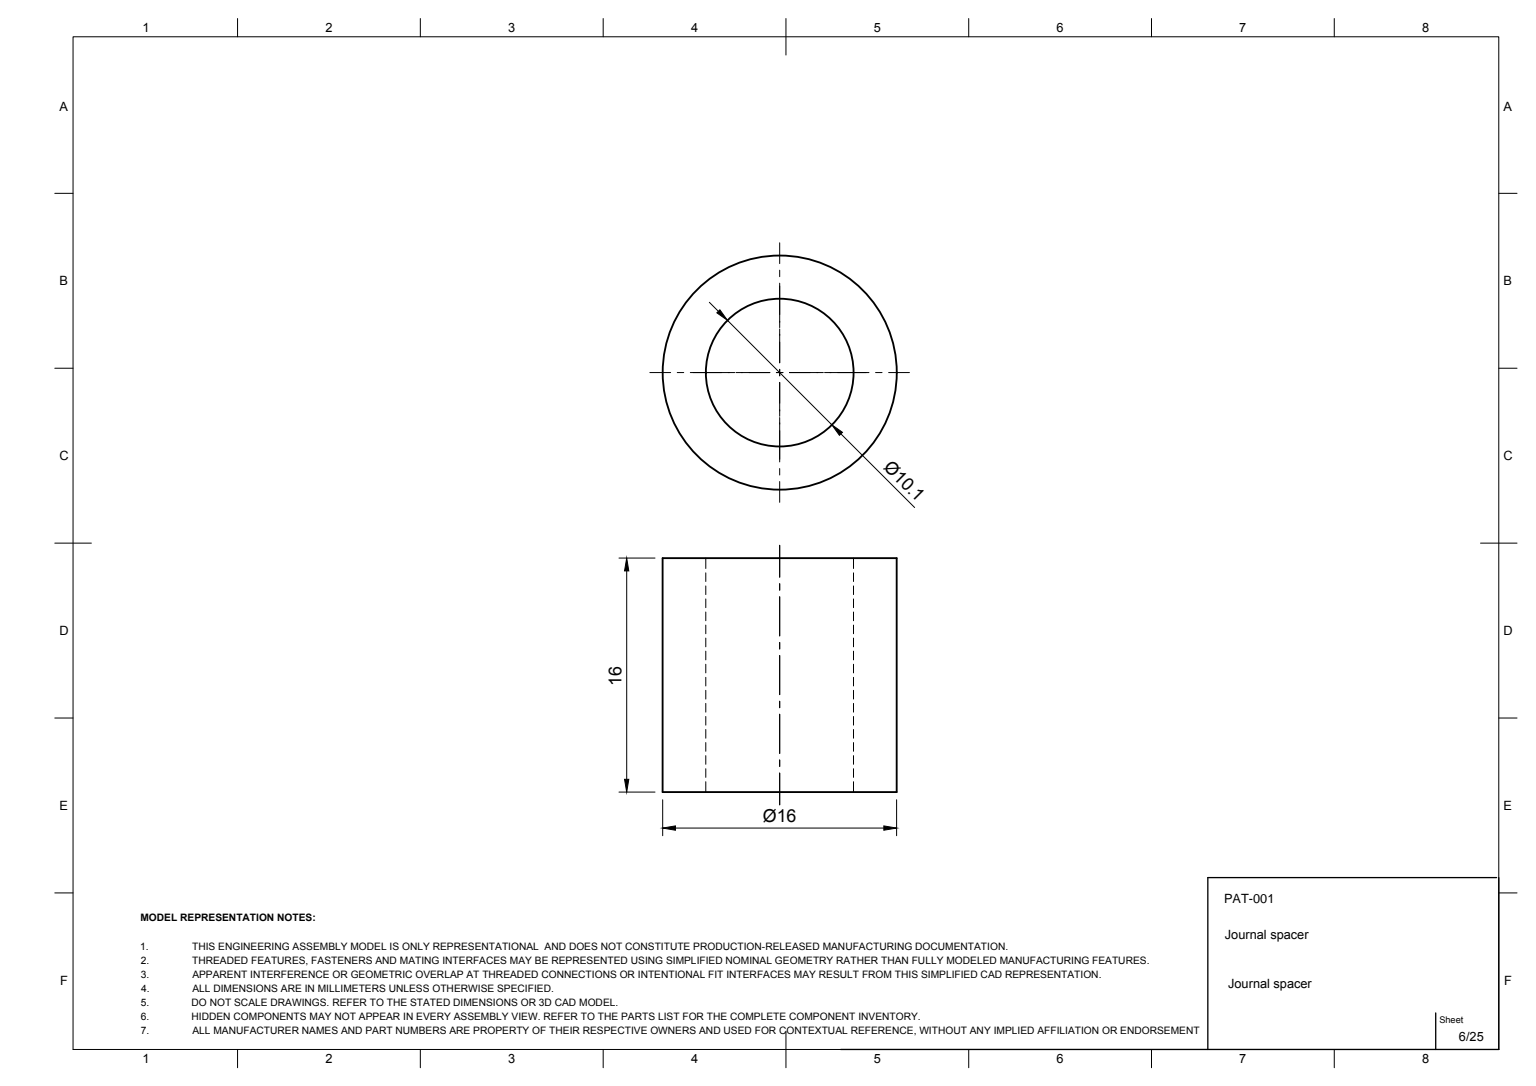
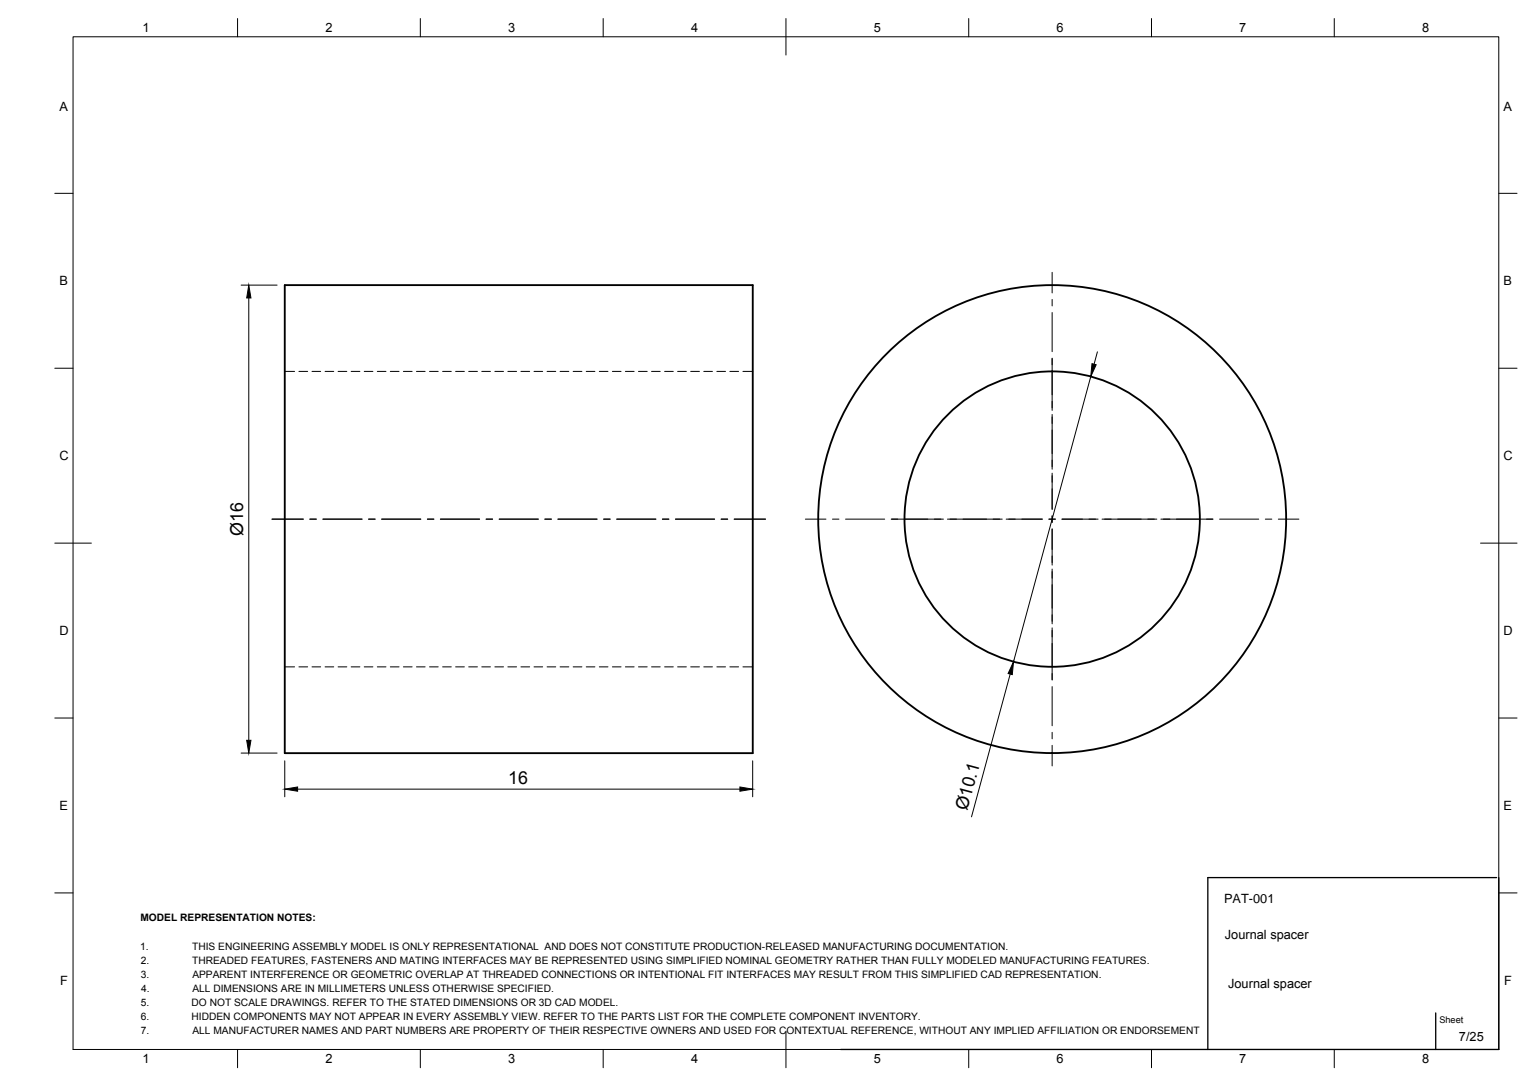
ISO-10303-21;
HEADER;
/* Generated by software containing ST-Developer
 * from STEP Tools, Inc. (www.steptools.com) 
 */

FILE_DESCRIPTION(
/* description */ ('PAT-001'),
/* implementation_level */ '2;1');

FILE_NAME(
/* name */ 'Journal spacer.step',
/* time_stamp */ '2026-10-29T17:07:15-07:00',
/* author */ (''),
/* organization */ (''),
/* preprocessor_version */ 'ST-DEVELOPER v20.2',
/* originating_system */ 'Autodesk Translation Framework v15.17.0.0',
/* authorisation */ '');

FILE_SCHEMA (('AUTOMOTIVE_DESIGN { 1 0 10303 214 3 1 1 }'));
ENDSEC;

DATA;
#10=MECHANICAL_DESIGN_GEOMETRIC_PRESENTATION_REPRESENTATION('',(#374),#9622);
#324=SHAPE_REPRESENTATION_RELATIONSHIP('SRR','None',#9747,#349);
#349=ADVANCED_BREP_SHAPE_REPRESENTATION('',(#407),#9596);
#374=STYLED_ITEM('',(#9955),#407);
#407=MANIFOLD_SOLID_BREP('Body1',#5199);
#441=FACE_BOUND('',#1029,.T.);
#442=FACE_BOUND('',#1031,.T.);
#534=PLANE('',#5540);
#535=PLANE('',#5541);
#726=FACE_OUTER_BOUND('',#1026,.T.);
#727=FACE_OUTER_BOUND('',#1027,.T.);
#728=FACE_OUTER_BOUND('',#1028,.T.);
#729=FACE_OUTER_BOUND('',#1030,.T.);
#1026=EDGE_LOOP('',(#3547,#3548,#3549,#3550));
#1027=EDGE_LOOP('',(#3551,#3552,#3553,#3554));
#1028=EDGE_LOOP('',(#3555));
#1029=EDGE_LOOP('',(#3556));
#1030=EDGE_LOOP('',(#3557));
#1031=EDGE_LOOP('',(#3558));
#1403=LINE('',#7752,#1808);
#1404=LINE('',#7758,#1809);
#1808=VECTOR('',#6166,0.505);
#1809=VECTOR('',#6173,0.8);
#2218=CIRCLE('',#5535,0.505);
#2219=CIRCLE('',#5536,0.505);
#2220=CIRCLE('',#5538,0.8);
#2221=CIRCLE('',#5539,0.8);
#2430=VERTEX_POINT('',#7749);
#2431=VERTEX_POINT('',#7751);
#2432=VERTEX_POINT('',#7755);
#2433=VERTEX_POINT('',#7757);
#2877=EDGE_CURVE('',#2430,#2430,#2218,.T.);
#2878=EDGE_CURVE('',#2430,#2431,#1403,.T.);
#2879=EDGE_CURVE('',#2431,#2431,#2219,.T.);
#2880=EDGE_CURVE('',#2432,#2432,#2220,.T.);
#2881=EDGE_CURVE('',#2432,#2433,#1404,.T.);
#2882=EDGE_CURVE('',#2433,#2433,#2221,.T.);
#3547=ORIENTED_EDGE('',*,*,#2877,.F.);
#3548=ORIENTED_EDGE('',*,*,#2878,.T.);
#3549=ORIENTED_EDGE('',*,*,#2879,.T.);
#3550=ORIENTED_EDGE('',*,*,#2878,.F.);
#3551=ORIENTED_EDGE('',*,*,#2880,.F.);
#3552=ORIENTED_EDGE('',*,*,#2881,.T.);
#3553=ORIENTED_EDGE('',*,*,#2882,.T.);
#3554=ORIENTED_EDGE('',*,*,#2881,.F.);
#3555=ORIENTED_EDGE('',*,*,#2880,.T.);
#3556=ORIENTED_EDGE('',*,*,#2877,.T.);
#3557=ORIENTED_EDGE('',*,*,#2882,.F.);
#3558=ORIENTED_EDGE('',*,*,#2879,.F.);
#4832=CYLINDRICAL_SURFACE('',#5534,0.505);
#4833=CYLINDRICAL_SURFACE('',#5537,0.8);
#4913=ADVANCED_FACE('',(#726),#4832,.F.);
#4914=ADVANCED_FACE('',(#727),#4833,.T.);
#4915=ADVANCED_FACE('',(#728,#441),#534,.T.);
#4916=ADVANCED_FACE('',(#729,#442),#535,.F.);
#5199=CLOSED_SHELL('',(#4913,#4914,#4915,#4916));
#5533=AXIS2_PLACEMENT_3D('',#7747,#6160,#6161);
#5534=AXIS2_PLACEMENT_3D('',#7748,#6162,#6163);
#5535=AXIS2_PLACEMENT_3D('',#7750,#6164,#6165);
#5536=AXIS2_PLACEMENT_3D('',#7753,#6167,#6168);
#5537=AXIS2_PLACEMENT_3D('',#7754,#6169,#6170);
#5538=AXIS2_PLACEMENT_3D('',#7756,#6171,#6172);
#5539=AXIS2_PLACEMENT_3D('',#7759,#6174,#6175);
#5540=AXIS2_PLACEMENT_3D('',#7760,#6176,#6177);
#5541=AXIS2_PLACEMENT_3D('',#7761,#6178,#6179);
#6160=DIRECTION('axis',(0.,0.,1.));
#6161=DIRECTION('refdir',(1.,0.,0.));
#6162=DIRECTION('center_axis',(0.,1.,0.));
#6163=DIRECTION('ref_axis',(1.,0.,0.));
#6164=DIRECTION('center_axis',(0.,-1.,0.));
#6165=DIRECTION('ref_axis',(1.,0.,0.));
#6166=DIRECTION('',(0.,-1.,0.));
#6167=DIRECTION('center_axis',(0.,-1.,0.));
#6168=DIRECTION('ref_axis',(1.,0.,0.));
#6169=DIRECTION('center_axis',(0.,1.,0.));
#6170=DIRECTION('ref_axis',(1.,0.,0.));
#6171=DIRECTION('center_axis',(0.,1.,0.));
#6172=DIRECTION('ref_axis',(1.,0.,0.));
#6173=DIRECTION('',(0.,-1.,0.));
#6174=DIRECTION('center_axis',(0.,1.,0.));
#6175=DIRECTION('ref_axis',(1.,0.,0.));
#6176=DIRECTION('center_axis',(0.,1.,0.));
#6177=DIRECTION('ref_axis',(1.,0.,0.));
#6178=DIRECTION('center_axis',(0.,1.,0.));
#6179=DIRECTION('ref_axis',(1.,0.,0.));
#7747=CARTESIAN_POINT('',(0.,0.,0.));
#7748=CARTESIAN_POINT('Origin',(0.,-1.6,4.5));
#7749=CARTESIAN_POINT('',(-0.505,0.,4.5));
#7750=CARTESIAN_POINT('Origin',(0.,0.,4.5));
#7751=CARTESIAN_POINT('',(-0.505,-1.6,4.5));
#7752=CARTESIAN_POINT('',(-0.505,-1.6,4.5));
#7753=CARTESIAN_POINT('Origin',(0.,-1.6,4.5));
#7754=CARTESIAN_POINT('Origin',(0.,-1.6,4.5));
#7755=CARTESIAN_POINT('',(-0.8,0.,4.5));
#7756=CARTESIAN_POINT('Origin',(0.,0.,4.5));
#7757=CARTESIAN_POINT('',(-0.8,-1.6,4.5));
#7758=CARTESIAN_POINT('',(-0.8,-1.6,4.5));
#7759=CARTESIAN_POINT('Origin',(0.,-1.6,4.5));
#7760=CARTESIAN_POINT('Origin',(0.,0.,4.5));
#7761=CARTESIAN_POINT('Origin',(0.,-1.6,4.5));
#9566=UNCERTAINTY_MEASURE_WITH_UNIT(LENGTH_MEASURE(0.001),#9623,
'DISTANCE_ACCURACY_VALUE',
'Maximum model space distance between geometric entities at asserted c
onnectivities');
#9592=UNCERTAINTY_MEASURE_WITH_UNIT(LENGTH_MEASURE(0.001),#9623,
'DISTANCE_ACCURACY_VALUE',
'Maximum model space distance between geometric entities at asserted c
onnectivities');
#9596=(
GEOMETRIC_REPRESENTATION_CONTEXT(3)
GLOBAL_UNCERTAINTY_ASSIGNED_CONTEXT((#9566))
GLOBAL_UNIT_ASSIGNED_CONTEXT((#9623,#9625,#9626))
REPRESENTATION_CONTEXT('','3D')
);
#9622=(
GEOMETRIC_REPRESENTATION_CONTEXT(3)
GLOBAL_UNCERTAINTY_ASSIGNED_CONTEXT((#9592))
GLOBAL_UNIT_ASSIGNED_CONTEXT((#9623,#9625,#9626))
REPRESENTATION_CONTEXT('','3D')
);
#9623=(
LENGTH_UNIT()
NAMED_UNIT(*)
SI_UNIT(.CENTI.,.METRE.)
);
#9625=(
NAMED_UNIT(*)
PLANE_ANGLE_UNIT()
SI_UNIT($,.RADIAN.)
);
#9626=(
NAMED_UNIT(*)
SI_UNIT($,.STERADIAN.)
SOLID_ANGLE_UNIT()
);
#9630=SHAPE_DEFINITION_REPRESENTATION(#9659,#9747);
#9659=PRODUCT_DEFINITION_SHAPE('',$,#9777);
#9747=SHAPE_REPRESENTATION('',(#5533),#9596);
#9773=PRODUCT_DEFINITION_CONTEXT('part definition',#9862,'design');
#9777=PRODUCT_DEFINITION('Journal spacer','Journal spacer',#9806,#9773);
#9806=PRODUCT_DEFINITION_FORMATION('',$,#9867);
#9862=APPLICATION_CONTEXT(
'Core Data for Automotive Mechanical Design Process');
#9863=PRODUCT_CONTEXT('part definition',#9862,'mechanical');
#9867=PRODUCT('Journal spacer','Journal spacer','Journal spacer',(#9863));
#9949=COLOUR_RGB('Sky Blue',0.24,0.69,0.87);
#9950=FILL_AREA_STYLE_COLOUR('',#9949);
#9951=FILL_AREA_STYLE('',(#9950));
#9952=SURFACE_STYLE_FILL_AREA(#9951);
#9953=SURFACE_SIDE_STYLE('',(#9952));
#9954=SURFACE_STYLE_USAGE(.BOTH.,#9953);
#9955=PRESENTATION_STYLE_ASSIGNMENT((#9954));
ENDSEC;
END-ISO-10303-21;
